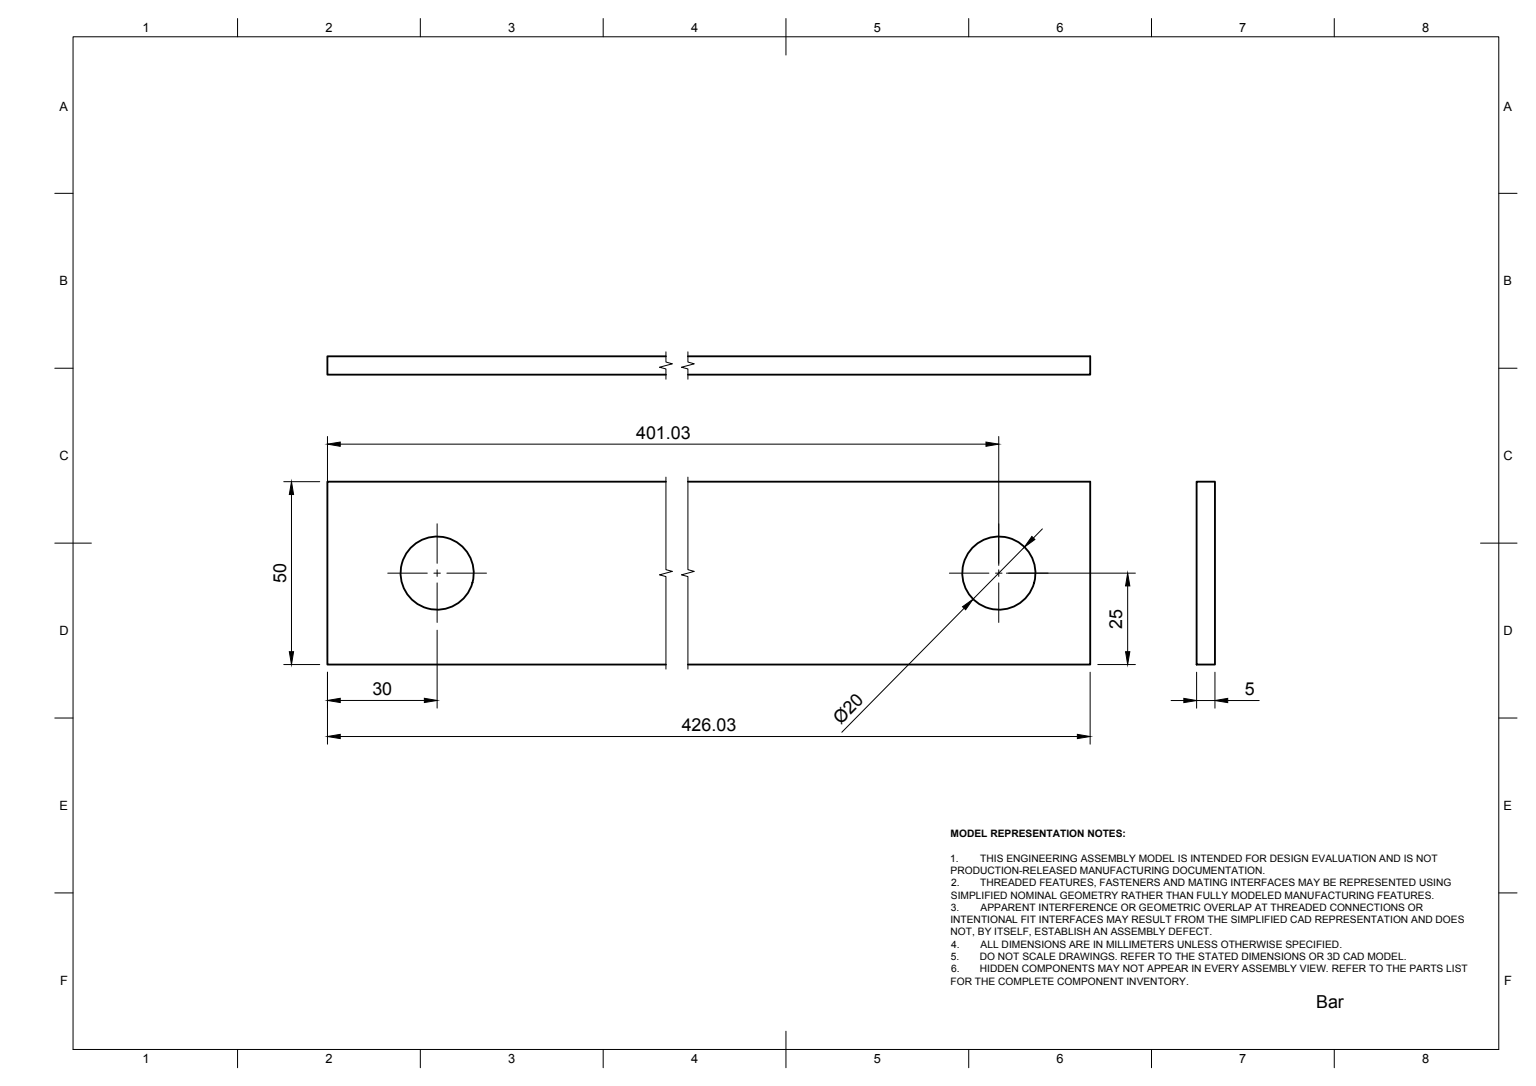
ISO-10303-21;
HEADER;
/* Generated by software containing ST-Developer
 * from STEP Tools, Inc. (www.steptools.com) 
 */

FILE_DESCRIPTION(
/* description */ (''),
/* implementation_level */ '2;1');

FILE_NAME(
/* name */ 'Bar.step',
/* time_stamp */ '2026-10-05T19:45:59-07:00',
/* author */ (''),
/* organization */ (''),
/* preprocessor_version */ 'ST-DEVELOPER v20.2',
/* originating_system */ 'Autodesk Translation Framework v15.15.0.0',
/* authorisation */ '');

FILE_SCHEMA (('AUTOMOTIVE_DESIGN { 1 0 10303 214 3 1 1 }'));
ENDSEC;

DATA;
#10=MECHANICAL_DESIGN_GEOMETRIC_PRESENTATION_REPRESENTATION('',(#94),#2462);
#61=FACE_BOUND('',#285,.T.);
#62=FACE_BOUND('',#286,.T.);
#63=FACE_BOUND('',#288,.T.);
#64=FACE_BOUND('',#289,.T.);
#76=SHAPE_REPRESENTATION_RELATIONSHIP('SRR','None',#2502,#85);
#85=ADVANCED_BREP_SHAPE_REPRESENTATION('',(#103),#2457);
#94=STYLED_ITEM('',(#2552),#103);
#103=MANIFOLD_SOLID_BREP('Body1',#1331);
#128=PLANE('',#1495);
#129=PLANE('',#1496);
#130=PLANE('',#1497);
#131=PLANE('',#1498);
#132=PLANE('',#1499);
#133=PLANE('',#1500);
#194=FACE_OUTER_BOUND('',#278,.T.);
#195=FACE_OUTER_BOUND('',#279,.T.);
#196=FACE_OUTER_BOUND('',#280,.T.);
#197=FACE_OUTER_BOUND('',#281,.T.);
#198=FACE_OUTER_BOUND('',#282,.T.);
#199=FACE_OUTER_BOUND('',#283,.T.);
#200=FACE_OUTER_BOUND('',#284,.T.);
#201=FACE_OUTER_BOUND('',#287,.T.);
#278=EDGE_LOOP('',(#1008,#1009,#1010,#1011));
#279=EDGE_LOOP('',(#1012,#1013,#1014,#1015));
#280=EDGE_LOOP('',(#1016,#1017,#1018,#1019));
#281=EDGE_LOOP('',(#1020,#1021,#1022,#1023));
#282=EDGE_LOOP('',(#1024,#1025,#1026,#1027));
#283=EDGE_LOOP('',(#1028,#1029,#1030,#1031));
#284=EDGE_LOOP('',(#1032,#1033,#1034,#1035));
#285=EDGE_LOOP('',(#1036));
#286=EDGE_LOOP('',(#1037));
#287=EDGE_LOOP('',(#1038,#1039,#1040,#1041));
#288=EDGE_LOOP('',(#1042));
#289=EDGE_LOOP('',(#1043));
#379=LINE('',#2118,#498);
#380=LINE('',#2124,#499);
#381=LINE('',#2129,#500);
#382=LINE('',#2131,#501);
#383=LINE('',#2133,#502);
#384=LINE('',#2134,#503);
#385=LINE('',#2137,#504);
#386=LINE('',#2139,#505);
#387=LINE('',#2140,#506);
#388=LINE('',#2143,#507);
#389=LINE('',#2145,#508);
#390=LINE('',#2146,#509);
#391=LINE('',#2148,#510);
#392=LINE('',#2149,#511);
#498=VECTOR('',#1728,10.);
#499=VECTOR('',#1735,10.);
#500=VECTOR('',#1740,10.);
#501=VECTOR('',#1741,10.);
#502=VECTOR('',#1742,10.);
#503=VECTOR('',#1743,10.);
#504=VECTOR('',#1746,10.);
#505=VECTOR('',#1747,10.);
#506=VECTOR('',#1748,10.);
#507=VECTOR('',#1751,10.);
#508=VECTOR('',#1752,10.);
#509=VECTOR('',#1753,10.);
#510=VECTOR('',#1756,10.);
#511=VECTOR('',#1757,10.);
#596=CIRCLE('',#1490,10.);
#597=CIRCLE('',#1491,10.);
#598=CIRCLE('',#1493,10.);
#599=CIRCLE('',#1494,10.);
#659=VERTEX_POINT('',#2115);
#660=VERTEX_POINT('',#2117);
#661=VERTEX_POINT('',#2121);
#662=VERTEX_POINT('',#2123);
#663=VERTEX_POINT('',#2127);
#664=VERTEX_POINT('',#2128);
#665=VERTEX_POINT('',#2130);
#666=VERTEX_POINT('',#2132);
#667=VERTEX_POINT('',#2136);
#668=VERTEX_POINT('',#2138);
#669=VERTEX_POINT('',#2142);
#670=VERTEX_POINT('',#2144);
#785=EDGE_CURVE('',#659,#659,#596,.T.);
#786=EDGE_CURVE('',#659,#660,#379,.T.);
#787=EDGE_CURVE('',#660,#660,#597,.T.);
#788=EDGE_CURVE('',#661,#661,#598,.T.);
#789=EDGE_CURVE('',#661,#662,#380,.T.);
#790=EDGE_CURVE('',#662,#662,#599,.T.);
#791=EDGE_CURVE('',#663,#664,#381,.T.);
#792=EDGE_CURVE('',#663,#665,#382,.F.);
#793=EDGE_CURVE('',#666,#665,#383,.T.);
#794=EDGE_CURVE('',#664,#666,#384,.T.);
#795=EDGE_CURVE('',#667,#664,#385,.F.);
#796=EDGE_CURVE('',#668,#666,#386,.F.);
#797=EDGE_CURVE('',#667,#668,#387,.F.);
#798=EDGE_CURVE('',#669,#667,#388,.T.);
#799=EDGE_CURVE('',#670,#668,#389,.T.);
#800=EDGE_CURVE('',#669,#670,#390,.T.);
#801=EDGE_CURVE('',#663,#669,#391,.F.);
#802=EDGE_CURVE('',#665,#670,#392,.F.);
#1008=ORIENTED_EDGE('',*,*,#785,.F.);
#1009=ORIENTED_EDGE('',*,*,#786,.T.);
#1010=ORIENTED_EDGE('',*,*,#787,.F.);
#1011=ORIENTED_EDGE('',*,*,#786,.F.);
#1012=ORIENTED_EDGE('',*,*,#788,.F.);
#1013=ORIENTED_EDGE('',*,*,#789,.T.);
#1014=ORIENTED_EDGE('',*,*,#790,.F.);
#1015=ORIENTED_EDGE('',*,*,#789,.F.);
#1016=ORIENTED_EDGE('',*,*,#791,.F.);
#1017=ORIENTED_EDGE('',*,*,#792,.T.);
#1018=ORIENTED_EDGE('',*,*,#793,.F.);
#1019=ORIENTED_EDGE('',*,*,#794,.F.);
#1020=ORIENTED_EDGE('',*,*,#795,.T.);
#1021=ORIENTED_EDGE('',*,*,#794,.T.);
#1022=ORIENTED_EDGE('',*,*,#796,.F.);
#1023=ORIENTED_EDGE('',*,*,#797,.F.);
#1024=ORIENTED_EDGE('',*,*,#798,.T.);
#1025=ORIENTED_EDGE('',*,*,#797,.T.);
#1026=ORIENTED_EDGE('',*,*,#799,.F.);
#1027=ORIENTED_EDGE('',*,*,#800,.F.);
#1028=ORIENTED_EDGE('',*,*,#801,.T.);
#1029=ORIENTED_EDGE('',*,*,#800,.T.);
#1030=ORIENTED_EDGE('',*,*,#802,.F.);
#1031=ORIENTED_EDGE('',*,*,#792,.F.);
#1032=ORIENTED_EDGE('',*,*,#802,.T.);
#1033=ORIENTED_EDGE('',*,*,#799,.T.);
#1034=ORIENTED_EDGE('',*,*,#796,.T.);
#1035=ORIENTED_EDGE('',*,*,#793,.T.);
#1036=ORIENTED_EDGE('',*,*,#785,.T.);
#1037=ORIENTED_EDGE('',*,*,#788,.T.);
#1038=ORIENTED_EDGE('',*,*,#801,.F.);
#1039=ORIENTED_EDGE('',*,*,#791,.T.);
#1040=ORIENTED_EDGE('',*,*,#795,.F.);
#1041=ORIENTED_EDGE('',*,*,#798,.F.);
#1042=ORIENTED_EDGE('',*,*,#787,.T.);
#1043=ORIENTED_EDGE('',*,*,#790,.T.);
#1235=CYLINDRICAL_SURFACE('',#1489,10.);
#1236=CYLINDRICAL_SURFACE('',#1492,10.);
#1276=ADVANCED_FACE('',(#194),#1235,.F.);
#1277=ADVANCED_FACE('',(#195),#1236,.F.);
#1278=ADVANCED_FACE('',(#196),#128,.T.);
#1279=ADVANCED_FACE('',(#197),#129,.T.);
#1280=ADVANCED_FACE('',(#198),#130,.T.);
#1281=ADVANCED_FACE('',(#199),#131,.T.);
#1282=ADVANCED_FACE('',(#200,#61,#62),#132,.T.);
#1283=ADVANCED_FACE('',(#201,#63,#64),#133,.F.);
#1331=CLOSED_SHELL('',(#1276,#1277,#1278,#1279,#1280,#1281,#1282,#1283));
#1488=AXIS2_PLACEMENT_3D('',#2113,#1722,#1723);
#1489=AXIS2_PLACEMENT_3D('',#2114,#1724,#1725);
#1490=AXIS2_PLACEMENT_3D('',#2116,#1726,#1727);
#1491=AXIS2_PLACEMENT_3D('',#2119,#1729,#1730);
#1492=AXIS2_PLACEMENT_3D('',#2120,#1731,#1732);
#1493=AXIS2_PLACEMENT_3D('',#2122,#1733,#1734);
#1494=AXIS2_PLACEMENT_3D('',#2125,#1736,#1737);
#1495=AXIS2_PLACEMENT_3D('',#2126,#1738,#1739);
#1496=AXIS2_PLACEMENT_3D('',#2135,#1744,#1745);
#1497=AXIS2_PLACEMENT_3D('',#2141,#1749,#1750);
#1498=AXIS2_PLACEMENT_3D('',#2147,#1754,#1755);
#1499=AXIS2_PLACEMENT_3D('',#2150,#1758,#1759);
#1500=AXIS2_PLACEMENT_3D('',#2151,#1760,#1761);
#1722=DIRECTION('axis',(0.,0.,1.));
#1723=DIRECTION('refdir',(1.,0.,0.));
#1724=DIRECTION('center_axis',(0.,0.,-1.));
#1725=DIRECTION('ref_axis',(-1.,0.,0.));
#1726=DIRECTION('center_axis',(0.,0.,-1.));
#1727=DIRECTION('ref_axis',(-1.,0.,0.));
#1728=DIRECTION('',(0.,0.,-1.));
#1729=DIRECTION('center_axis',(0.,0.,1.));
#1730=DIRECTION('ref_axis',(-1.,0.,0.));
#1731=DIRECTION('center_axis',(0.,0.,-1.));
#1732=DIRECTION('ref_axis',(-1.,0.,0.));
#1733=DIRECTION('center_axis',(0.,0.,-1.));
#1734=DIRECTION('ref_axis',(-1.,0.,0.));
#1735=DIRECTION('',(0.,0.,-1.));
#1736=DIRECTION('center_axis',(0.,0.,1.));
#1737=DIRECTION('ref_axis',(-1.,0.,0.));
#1738=DIRECTION('center_axis',(-0.261435213626798,-0.965221026022491,0.));
#1739=DIRECTION('ref_axis',(0.965221026022491,-0.261435213626798,0.));
#1740=DIRECTION('',(-0.965221026022491,0.261435213626798,0.));
#1741=DIRECTION('',(0.,0.,-1.));
#1742=DIRECTION('',(0.965221026022491,-0.261435213626798,0.));
#1743=DIRECTION('',(0.,0.,1.));
#1744=DIRECTION('center_axis',(-0.965221026022491,0.261435213626798,0.));
#1745=DIRECTION('ref_axis',(-0.261435213626798,-0.965221026022491,0.));
#1746=DIRECTION('',(0.261435213626798,0.965221026022491,0.));
#1747=DIRECTION('',(0.261435213626798,0.965221026022491,0.));
#1748=DIRECTION('',(0.,0.,-1.));
#1749=DIRECTION('center_axis',(0.261435213626798,0.965221026022491,0.));
#1750=DIRECTION('ref_axis',(-0.965221026022491,0.261435213626798,0.));
#1751=DIRECTION('',(-0.965221026022491,0.261435213626798,0.));
#1752=DIRECTION('',(-0.965221026022491,0.261435213626798,0.));
#1753=DIRECTION('',(0.,0.,1.));
#1754=DIRECTION('center_axis',(0.965221026022491,-0.261435213626797,0.));
#1755=DIRECTION('ref_axis',(0.261435213626797,0.965221026022491,0.));
#1756=DIRECTION('',(-0.261435213626797,-0.965221026022491,0.));
#1757=DIRECTION('',(-0.261435213626797,-0.965221026022491,0.));
#1758=DIRECTION('center_axis',(0.,0.,1.));
#1759=DIRECTION('ref_axis',(1.,0.,0.));
#1760=DIRECTION('center_axis',(0.,0.,1.));
#1761=DIRECTION('ref_axis',(-1.,0.,0.));
#2113=CARTESIAN_POINT('',(0.,0.,0.));
#2114=CARTESIAN_POINT('Origin',(152.4,-2.52242671194836E-12,19.9999999999958));
#2115=CARTESIAN_POINT('',(162.4,-2.52120206514921E-12,19.9999999999958));
#2116=CARTESIAN_POINT('Origin',(152.4,-2.52242671194836E-12,19.9999999999958));
#2117=CARTESIAN_POINT('',(162.4,-2.52120206514921E-12,14.9999999999958));
#2118=CARTESIAN_POINT('',(162.4,-2.52365135874751E-12,19.9999999999958));
#2119=CARTESIAN_POINT('Origin',(152.4,-2.52242671194836E-12,14.9999999999958));
#2120=CARTESIAN_POINT('Origin',(-205.724822686805,97.,19.9999999999958));
#2121=CARTESIAN_POINT('',(-195.724822686805,97.,19.9999999999958));
#2122=CARTESIAN_POINT('Origin',(-205.724822686805,97.,19.9999999999958));
#2123=CARTESIAN_POINT('',(-195.724822686805,97.,14.9999999999958));
#2124=CARTESIAN_POINT('',(-195.724822686805,97.,19.9999999999958));
#2125=CARTESIAN_POINT('Origin',(-205.724822686805,97.,14.9999999999958));
#2126=CARTESIAN_POINT('Origin',(-212.260703027475,72.8694743494378,14.9999999999958));
#2127=CARTESIAN_POINT('',(169.994645309892,-30.6664059912348,14.9999999999958));
#2128=CARTESIAN_POINT('',(-241.21733380815,80.7125307582417,14.9999999999958));
#2129=CARTESIAN_POINT('',(145.86411965933,-24.1305256505648,14.9999999999958));
#2130=CARTESIAN_POINT('',(169.994645309892,-30.6664059912348,19.9999999999958));
#2131=CARTESIAN_POINT('',(169.994645309892,-30.6664059912348,14.9999999999958));
#2132=CARTESIAN_POINT('',(-241.21733380815,80.7125307582417,19.9999999999958));
#2133=CARTESIAN_POINT('',(145.86411965933,-24.1305256505648,19.9999999999958));
#2134=CARTESIAN_POINT('',(-241.21733380815,80.7125307582417,14.9999999999958));
#2135=CARTESIAN_POINT('Origin',(-228.14557312681,128.973582059366,14.9999999999958));
#2136=CARTESIAN_POINT('',(-228.14557312681,128.973582059366,14.9999999999958));
#2137=CARTESIAN_POINT('',(-231.413513297145,116.908319234085,14.9999999999958));
#2138=CARTESIAN_POINT('',(-228.14557312681,128.973582059366,19.9999999999958));
#2139=CARTESIAN_POINT('',(-231.413513297145,116.908319234085,19.9999999999958));
#2140=CARTESIAN_POINT('',(-228.14557312681,128.973582059366,14.9999999999958));
#2141=CARTESIAN_POINT('Origin',(158.93588034067,24.1305256505598,14.9999999999958));
#2142=CARTESIAN_POINT('',(183.066405991232,17.5946453098898,14.9999999999958));
#2143=CARTESIAN_POINT('',(158.93588034067,24.1305256505598,14.9999999999958));
#2144=CARTESIAN_POINT('',(183.066405991232,17.5946453098898,19.9999999999958));
#2145=CARTESIAN_POINT('',(158.93588034067,24.1305256505598,19.9999999999958));
#2146=CARTESIAN_POINT('',(183.066405991232,17.5946453098898,14.9999999999958));
#2147=CARTESIAN_POINT('Origin',(169.994645309892,-30.6664059912347,14.9999999999958));
#2148=CARTESIAN_POINT('',(173.262585480227,-18.6011431659535,14.9999999999958));
#2149=CARTESIAN_POINT('',(173.262585480227,-18.6011431659535,19.9999999999958));
#2150=CARTESIAN_POINT('Origin',(-26.6624113434025,48.4999999999987,19.9999999999958));
#2151=CARTESIAN_POINT('Origin',(-26.6624113434025,48.4999999999987,14.9999999999958));
#2446=UNCERTAINTY_MEASURE_WITH_UNIT(LENGTH_MEASURE(0.01),#2463,
'DISTANCE_ACCURACY_VALUE',
'Maximum model space distance between geometric entities at asserted c
onnectivities');
#2451=UNCERTAINTY_MEASURE_WITH_UNIT(LENGTH_MEASURE(0.01),#2463,
'DISTANCE_ACCURACY_VALUE',
'Maximum model space distance between geometric entities at asserted c
onnectivities');
#2457=(
GEOMETRIC_REPRESENTATION_CONTEXT(3)
GLOBAL_UNCERTAINTY_ASSIGNED_CONTEXT((#2446))
GLOBAL_UNIT_ASSIGNED_CONTEXT((#2463,#2465,#2466))
REPRESENTATION_CONTEXT('','3D')
);
#2462=(
GEOMETRIC_REPRESENTATION_CONTEXT(3)
GLOBAL_UNCERTAINTY_ASSIGNED_CONTEXT((#2451))
GLOBAL_UNIT_ASSIGNED_CONTEXT((#2463,#2465,#2466))
REPRESENTATION_CONTEXT('','3D')
);
#2463=(
LENGTH_UNIT()
NAMED_UNIT(*)
SI_UNIT(.MILLI.,.METRE.)
);
#2465=(
NAMED_UNIT(*)
PLANE_ANGLE_UNIT()
SI_UNIT($,.RADIAN.)
);
#2466=(
NAMED_UNIT(*)
SI_UNIT($,.STERADIAN.)
SOLID_ANGLE_UNIT()
);
#2472=SHAPE_DEFINITION_REPRESENTATION(#2482,#2502);
#2482=PRODUCT_DEFINITION_SHAPE('',$,#2513);
#2502=SHAPE_REPRESENTATION('',(#1488),#2457);
#2507=PRODUCT_DEFINITION_CONTEXT('part definition',#2539,'design');
#2513=PRODUCT_DEFINITION('Bar','Bar',#2523,#2507);
#2523=PRODUCT_DEFINITION_FORMATION('',$,#2546);
#2539=APPLICATION_CONTEXT(
'Core Data for Automotive Mechanical Design Process');
#2540=PRODUCT_CONTEXT('part definition',#2539,'mechanical');
#2546=PRODUCT('Bar','Bar',$,(#2540));
#2552=PRESENTATION_STYLE_ASSIGNMENT((#2555));
#2555=SURFACE_STYLE_USAGE(.BOTH.,#2558);
#2558=SURFACE_SIDE_STYLE('',(#2561));
#2561=SURFACE_STYLE_FILL_AREA(#2564);
#2564=FILL_AREA_STYLE('Opaque(160,160,160)',(#2567));
#2567=FILL_AREA_STYLE_COLOUR('Opaque(160,160,160)',#2570);
#2570=COLOUR_RGB('Opaque(160,160,160)', 0.09019608, 0.27058824, 0.51372549);
ENDSEC;
END-ISO-10303-21;
